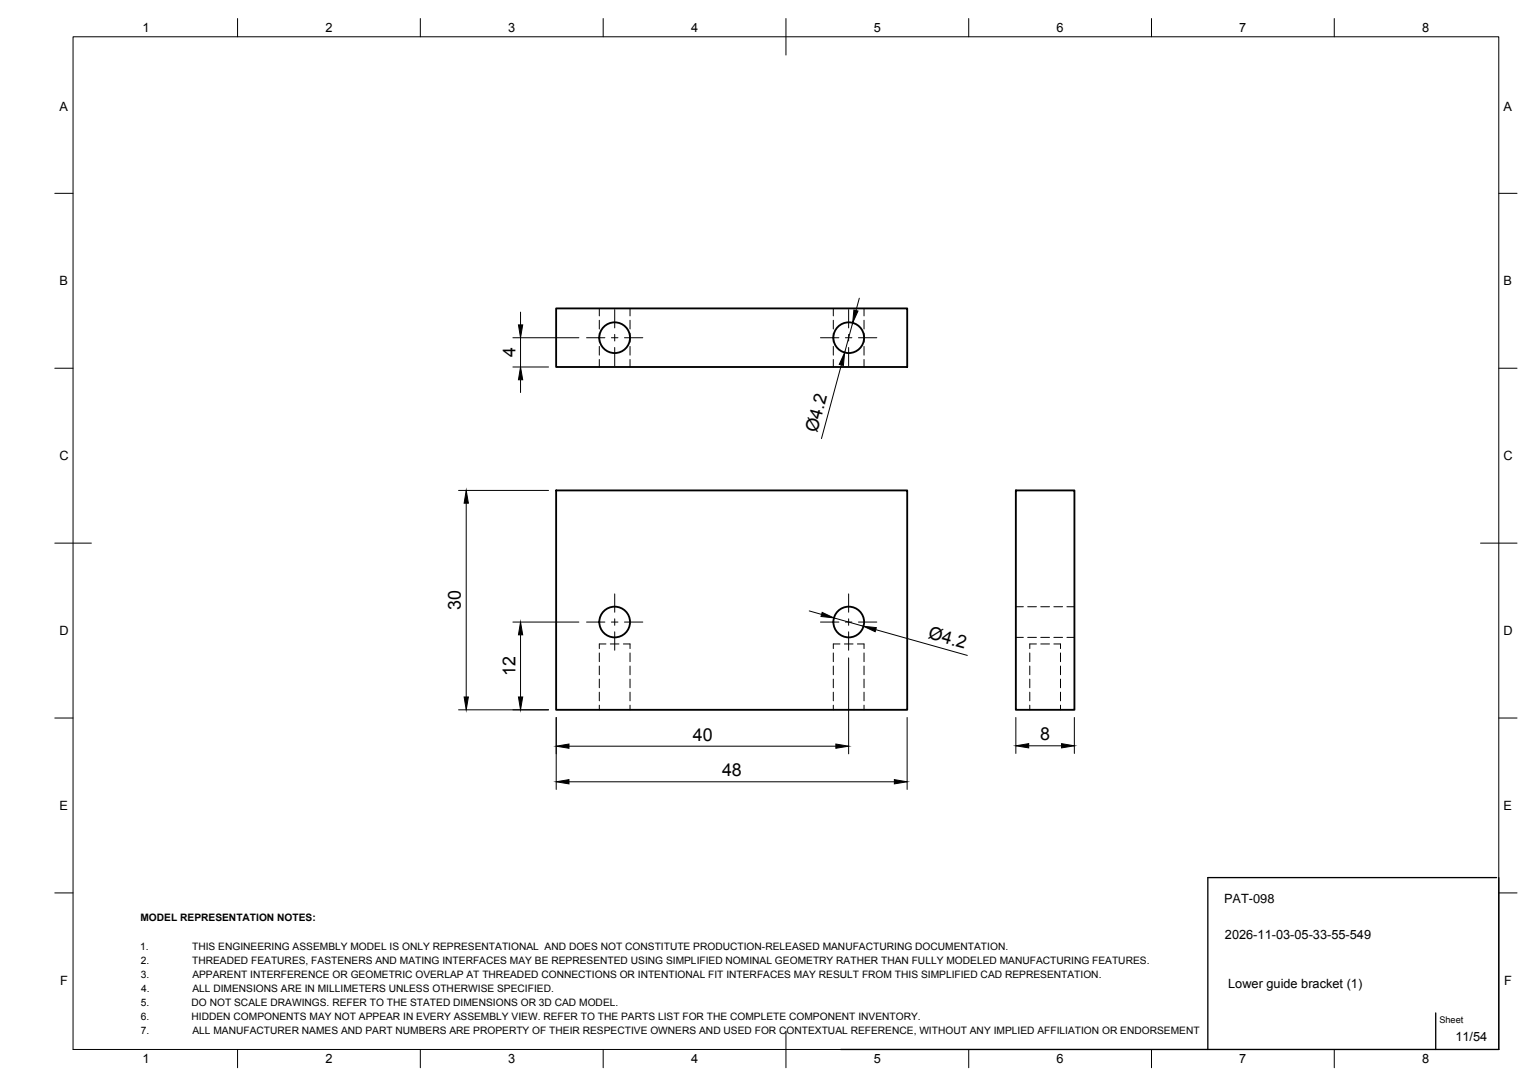
ISO-10303-21;
HEADER;
/* Generated by software containing ST-Developer
 * from STEP Tools, Inc. (www.steptools.com) 
 */

FILE_DESCRIPTION(
/* description */ ('Spring compression tester'),
/* implementation_level */ '2;1');

FILE_NAME(
/* name */ 'Lower guide bracket (1).step',
/* time_stamp */ '2026-10-28T03:24:11-07:00',
/* author */ (''),
/* organization */ (''),
/* preprocessor_version */ 'ST-DEVELOPER v20.2',
/* originating_system */ 'Autodesk Translation Framework v15.17.0.0',
/* authorisation */ '');

FILE_SCHEMA (('AUTOMOTIVE_DESIGN { 1 0 10303 214 3 1 1 }'));
ENDSEC;

DATA;
#10=MECHANICAL_DESIGN_GEOMETRIC_PRESENTATION_REPRESENTATION('',(#1112),#43521);
#992=SHAPE_REPRESENTATION_RELATIONSHIP('SRR','None',#43804,#1052);
#1052=ADVANCED_BREP_SHAPE_REPRESENTATION('',(#1187),#43464);
#1112=STYLED_ITEM('',(#44181),#1187);
#1187=MANIFOLD_SOLID_BREP('Body1',#18549);
#1333=FACE_BOUND('',#3434,.T.);
#1334=FACE_BOUND('',#3435,.T.);
#1335=FACE_BOUND('',#3438,.T.);
#1336=FACE_BOUND('',#3439,.T.);
#1337=FACE_BOUND('',#3443,.T.);
#1338=FACE_BOUND('',#3444,.T.);
#1663=PLANE('',#19526);
#1664=PLANE('',#19530);
#1665=PLANE('',#19537);
#1666=PLANE('',#19538);
#1667=PLANE('',#19539);
#1668=PLANE('',#19540);
#1669=PLANE('',#19541);
#1670=PLANE('',#19542);
#2294=FACE_OUTER_BOUND('',#3427,.T.);
#2295=FACE_OUTER_BOUND('',#3428,.T.);
#2296=FACE_OUTER_BOUND('',#3429,.T.);
#2297=FACE_OUTER_BOUND('',#3430,.T.);
#2298=FACE_OUTER_BOUND('',#3431,.T.);
#2299=FACE_OUTER_BOUND('',#3432,.T.);
#2300=FACE_OUTER_BOUND('',#3433,.T.);
#2301=FACE_OUTER_BOUND('',#3436,.T.);
#2302=FACE_OUTER_BOUND('',#3437,.T.);
#2303=FACE_OUTER_BOUND('',#3440,.T.);
#2304=FACE_OUTER_BOUND('',#3441,.T.);
#2305=FACE_OUTER_BOUND('',#3442,.T.);
#3427=EDGE_LOOP('',(#12793,#12794,#12795,#12796));
#3428=EDGE_LOOP('',(#12797));
#3429=EDGE_LOOP('',(#12798,#12799,#12800,#12801));
#3430=EDGE_LOOP('',(#12802));
#3431=EDGE_LOOP('',(#12803,#12804,#12805,#12806));
#3432=EDGE_LOOP('',(#12807,#12808,#12809,#12810));
#3433=EDGE_LOOP('',(#12811,#12812,#12813,#12814));
#3434=EDGE_LOOP('',(#12815));
#3435=EDGE_LOOP('',(#12816));
#3436=EDGE_LOOP('',(#12817,#12818,#12819,#12820));
#3437=EDGE_LOOP('',(#12821,#12822,#12823,#12824));
#3438=EDGE_LOOP('',(#12825));
#3439=EDGE_LOOP('',(#12826));
#3440=EDGE_LOOP('',(#12827,#12828,#12829,#12830));
#3441=EDGE_LOOP('',(#12831,#12832,#12833,#12834));
#3442=EDGE_LOOP('',(#12835,#12836,#12837,#12838));
#3443=EDGE_LOOP('',(#12839));
#3444=EDGE_LOOP('',(#12840));
#4790=LINE('',#27071,#6222);
#4791=LINE('',#27078,#6223);
#4792=LINE('',#27085,#6224);
#4793=LINE('',#27091,#6225);
#4794=LINE('',#27096,#6226);
#4795=LINE('',#27098,#6227);
#4796=LINE('',#27100,#6228);
#4797=LINE('',#27101,#6229);
#4798=LINE('',#27104,#6230);
#4799=LINE('',#27106,#6231);
#4800=LINE('',#27107,#6232);
#4801=LINE('',#27110,#6233);
#4802=LINE('',#27112,#6234);
#4803=LINE('',#27113,#6235);
#4804=LINE('',#27115,#6236);
#4805=LINE('',#27116,#6237);
#6222=VECTOR('',#21862,0.21);
#6223=VECTOR('',#21871,0.21);
#6224=VECTOR('',#21880,0.21);
#6225=VECTOR('',#21887,0.21);
#6226=VECTOR('',#21892,1.);
#6227=VECTOR('',#21893,1.);
#6228=VECTOR('',#21894,1.);
#6229=VECTOR('',#21895,1.);
#6230=VECTOR('',#21898,1.);
#6231=VECTOR('',#21899,1.);
#6232=VECTOR('',#21900,1.);
#6233=VECTOR('',#21903,1.);
#6234=VECTOR('',#21904,1.);
#6235=VECTOR('',#21905,1.);
#6236=VECTOR('',#21908,1.);
#6237=VECTOR('',#21909,1.);
#7574=CIRCLE('',#19524,0.21);
#7575=CIRCLE('',#19525,0.21);
#7576=CIRCLE('',#19528,0.21);
#7577=CIRCLE('',#19529,0.21);
#7578=CIRCLE('',#19532,0.21);
#7579=CIRCLE('',#19533,0.21);
#7580=CIRCLE('',#19535,0.21);
#7581=CIRCLE('',#19536,0.21);
#8328=VERTEX_POINT('',#27068);
#8329=VERTEX_POINT('',#27070);
#8330=VERTEX_POINT('',#27075);
#8331=VERTEX_POINT('',#27077);
#8332=VERTEX_POINT('',#27082);
#8333=VERTEX_POINT('',#27084);
#8334=VERTEX_POINT('',#27088);
#8335=VERTEX_POINT('',#27090);
#8336=VERTEX_POINT('',#27094);
#8337=VERTEX_POINT('',#27095);
#8338=VERTEX_POINT('',#27097);
#8339=VERTEX_POINT('',#27099);
#8340=VERTEX_POINT('',#27103);
#8341=VERTEX_POINT('',#27105);
#8342=VERTEX_POINT('',#27109);
#8343=VERTEX_POINT('',#27111);
#10061=EDGE_CURVE('',#8328,#8328,#7574,.T.);
#10062=EDGE_CURVE('',#8328,#8329,#4790,.T.);
#10063=EDGE_CURVE('',#8329,#8329,#7575,.T.);
#10064=EDGE_CURVE('',#8330,#8330,#7576,.T.);
#10065=EDGE_CURVE('',#8330,#8331,#4791,.T.);
#10066=EDGE_CURVE('',#8331,#8331,#7577,.T.);
#10067=EDGE_CURVE('',#8332,#8332,#7578,.T.);
#10068=EDGE_CURVE('',#8332,#8333,#4792,.T.);
#10069=EDGE_CURVE('',#8333,#8333,#7579,.T.);
#10070=EDGE_CURVE('',#8334,#8334,#7580,.T.);
#10071=EDGE_CURVE('',#8334,#8335,#4793,.T.);
#10072=EDGE_CURVE('',#8335,#8335,#7581,.T.);
#10073=EDGE_CURVE('',#8336,#8337,#4794,.T.);
#10074=EDGE_CURVE('',#8337,#8338,#4795,.T.);
#10075=EDGE_CURVE('',#8339,#8338,#4796,.T.);
#10076=EDGE_CURVE('',#8336,#8339,#4797,.T.);
#10077=EDGE_CURVE('',#8340,#8336,#4798,.T.);
#10078=EDGE_CURVE('',#8341,#8339,#4799,.T.);
#10079=EDGE_CURVE('',#8340,#8341,#4800,.T.);
#10080=EDGE_CURVE('',#8342,#8340,#4801,.T.);
#10081=EDGE_CURVE('',#8343,#8341,#4802,.T.);
#10082=EDGE_CURVE('',#8342,#8343,#4803,.T.);
#10083=EDGE_CURVE('',#8337,#8342,#4804,.T.);
#10084=EDGE_CURVE('',#8338,#8343,#4805,.T.);
#12793=ORIENTED_EDGE('',*,*,#10061,.F.);
#12794=ORIENTED_EDGE('',*,*,#10062,.T.);
#12795=ORIENTED_EDGE('',*,*,#10063,.T.);
#12796=ORIENTED_EDGE('',*,*,#10062,.F.);
#12797=ORIENTED_EDGE('',*,*,#10063,.F.);
#12798=ORIENTED_EDGE('',*,*,#10064,.F.);
#12799=ORIENTED_EDGE('',*,*,#10065,.T.);
#12800=ORIENTED_EDGE('',*,*,#10066,.T.);
#12801=ORIENTED_EDGE('',*,*,#10065,.F.);
#12802=ORIENTED_EDGE('',*,*,#10066,.F.);
#12803=ORIENTED_EDGE('',*,*,#10067,.F.);
#12804=ORIENTED_EDGE('',*,*,#10068,.T.);
#12805=ORIENTED_EDGE('',*,*,#10069,.F.);
#12806=ORIENTED_EDGE('',*,*,#10068,.F.);
#12807=ORIENTED_EDGE('',*,*,#10070,.F.);
#12808=ORIENTED_EDGE('',*,*,#10071,.T.);
#12809=ORIENTED_EDGE('',*,*,#10072,.F.);
#12810=ORIENTED_EDGE('',*,*,#10071,.F.);
#12811=ORIENTED_EDGE('',*,*,#10073,.T.);
#12812=ORIENTED_EDGE('',*,*,#10074,.T.);
#12813=ORIENTED_EDGE('',*,*,#10075,.F.);
#12814=ORIENTED_EDGE('',*,*,#10076,.F.);
#12815=ORIENTED_EDGE('',*,*,#10069,.T.);
#12816=ORIENTED_EDGE('',*,*,#10072,.T.);
#12817=ORIENTED_EDGE('',*,*,#10077,.T.);
#12818=ORIENTED_EDGE('',*,*,#10076,.T.);
#12819=ORIENTED_EDGE('',*,*,#10078,.F.);
#12820=ORIENTED_EDGE('',*,*,#10079,.F.);
#12821=ORIENTED_EDGE('',*,*,#10080,.T.);
#12822=ORIENTED_EDGE('',*,*,#10079,.T.);
#12823=ORIENTED_EDGE('',*,*,#10081,.F.);
#12824=ORIENTED_EDGE('',*,*,#10082,.F.);
#12825=ORIENTED_EDGE('',*,*,#10067,.T.);
#12826=ORIENTED_EDGE('',*,*,#10070,.T.);
#12827=ORIENTED_EDGE('',*,*,#10083,.T.);
#12828=ORIENTED_EDGE('',*,*,#10082,.T.);
#12829=ORIENTED_EDGE('',*,*,#10084,.F.);
#12830=ORIENTED_EDGE('',*,*,#10074,.F.);
#12831=ORIENTED_EDGE('',*,*,#10084,.T.);
#12832=ORIENTED_EDGE('',*,*,#10081,.T.);
#12833=ORIENTED_EDGE('',*,*,#10078,.T.);
#12834=ORIENTED_EDGE('',*,*,#10075,.T.);
#12835=ORIENTED_EDGE('',*,*,#10083,.F.);
#12836=ORIENTED_EDGE('',*,*,#10073,.F.);
#12837=ORIENTED_EDGE('',*,*,#10077,.F.);
#12838=ORIENTED_EDGE('',*,*,#10080,.F.);
#12839=ORIENTED_EDGE('',*,*,#10061,.T.);
#12840=ORIENTED_EDGE('',*,*,#10064,.T.);
#17155=CYLINDRICAL_SURFACE('',#19523,0.21);
#17156=CYLINDRICAL_SURFACE('',#19527,0.21);
#17157=CYLINDRICAL_SURFACE('',#19531,0.21);
#17158=CYLINDRICAL_SURFACE('',#19534,0.21);
#17618=ADVANCED_FACE('',(#2294),#17155,.F.);
#17619=ADVANCED_FACE('',(#2295),#1663,.F.);
#17620=ADVANCED_FACE('',(#2296),#17156,.F.);
#17621=ADVANCED_FACE('',(#2297),#1664,.F.);
#17622=ADVANCED_FACE('',(#2298),#17157,.F.);
#17623=ADVANCED_FACE('',(#2299),#17158,.F.);
#17624=ADVANCED_FACE('',(#2300,#1333,#1334),#1665,.T.);
#17625=ADVANCED_FACE('',(#2301),#1666,.T.);
#17626=ADVANCED_FACE('',(#2302,#1335,#1336),#1667,.T.);
#17627=ADVANCED_FACE('',(#2303),#1668,.T.);
#17628=ADVANCED_FACE('',(#2304),#1669,.T.);
#17629=ADVANCED_FACE('',(#2305,#1337,#1338),#1670,.F.);
#18549=CLOSED_SHELL('',(#17618,#17619,#17620,#17621,#17622,#17623,#17624,
#17625,#17626,#17627,#17628,#17629));
#19522=AXIS2_PLACEMENT_3D('',#27066,#21856,#21857);
#19523=AXIS2_PLACEMENT_3D('',#27067,#21858,#21859);
#19524=AXIS2_PLACEMENT_3D('',#27069,#21860,#21861);
#19525=AXIS2_PLACEMENT_3D('',#27072,#21863,#21864);
#19526=AXIS2_PLACEMENT_3D('',#27073,#21865,#21866);
#19527=AXIS2_PLACEMENT_3D('',#27074,#21867,#21868);
#19528=AXIS2_PLACEMENT_3D('',#27076,#21869,#21870);
#19529=AXIS2_PLACEMENT_3D('',#27079,#21872,#21873);
#19530=AXIS2_PLACEMENT_3D('',#27080,#21874,#21875);
#19531=AXIS2_PLACEMENT_3D('',#27081,#21876,#21877);
#19532=AXIS2_PLACEMENT_3D('',#27083,#21878,#21879);
#19533=AXIS2_PLACEMENT_3D('',#27086,#21881,#21882);
#19534=AXIS2_PLACEMENT_3D('',#27087,#21883,#21884);
#19535=AXIS2_PLACEMENT_3D('',#27089,#21885,#21886);
#19536=AXIS2_PLACEMENT_3D('',#27092,#21888,#21889);
#19537=AXIS2_PLACEMENT_3D('',#27093,#21890,#21891);
#19538=AXIS2_PLACEMENT_3D('',#27102,#21896,#21897);
#19539=AXIS2_PLACEMENT_3D('',#27108,#21901,#21902);
#19540=AXIS2_PLACEMENT_3D('',#27114,#21906,#21907);
#19541=AXIS2_PLACEMENT_3D('',#27117,#21910,#21911);
#19542=AXIS2_PLACEMENT_3D('',#27118,#21912,#21913);
#21856=DIRECTION('axis',(0.,0.,1.));
#21857=DIRECTION('refdir',(1.,0.,0.));
#21858=DIRECTION('center_axis',(0.,0.,1.));
#21859=DIRECTION('ref_axis',(1.,0.,0.));
#21860=DIRECTION('center_axis',(0.,0.,1.));
#21861=DIRECTION('ref_axis',(1.,0.,0.));
#21862=DIRECTION('',(0.,0.,1.));
#21863=DIRECTION('center_axis',(0.,0.,1.));
#21864=DIRECTION('ref_axis',(1.,0.,0.));
#21865=DIRECTION('center_axis',(0.,0.,1.));
#21866=DIRECTION('ref_axis',(1.,0.,0.));
#21867=DIRECTION('center_axis',(0.,0.,1.));
#21868=DIRECTION('ref_axis',(1.,0.,0.));
#21869=DIRECTION('center_axis',(0.,0.,1.));
#21870=DIRECTION('ref_axis',(1.,0.,0.));
#21871=DIRECTION('',(0.,0.,1.));
#21872=DIRECTION('center_axis',(0.,0.,1.));
#21873=DIRECTION('ref_axis',(1.,0.,0.));
#21874=DIRECTION('center_axis',(0.,0.,1.));
#21875=DIRECTION('ref_axis',(1.,0.,0.));
#21876=DIRECTION('center_axis',(0.,1.,0.));
#21877=DIRECTION('ref_axis',(1.,0.,0.));
#21878=DIRECTION('center_axis',(0.,1.,0.));
#21879=DIRECTION('ref_axis',(1.,0.,0.));
#21880=DIRECTION('',(0.,1.,0.));
#21881=DIRECTION('center_axis',(0.,-1.,0.));
#21882=DIRECTION('ref_axis',(1.,0.,0.));
#21883=DIRECTION('center_axis',(0.,1.,0.));
#21884=DIRECTION('ref_axis',(1.,0.,0.));
#21885=DIRECTION('center_axis',(0.,1.,0.));
#21886=DIRECTION('ref_axis',(1.,0.,0.));
#21887=DIRECTION('',(0.,1.,0.));
#21888=DIRECTION('center_axis',(0.,-1.,0.));
#21889=DIRECTION('ref_axis',(1.,0.,0.));
#21890=DIRECTION('center_axis',(0.,1.,0.));
#21891=DIRECTION('ref_axis',(-1.,0.,0.));
#21892=DIRECTION('',(-1.,0.,0.));
#21893=DIRECTION('',(0.,0.,1.));
#21894=DIRECTION('',(-1.,0.,0.));
#21895=DIRECTION('',(0.,0.,1.));
#21896=DIRECTION('center_axis',(1.,0.,0.));
#21897=DIRECTION('ref_axis',(0.,1.,0.));
#21898=DIRECTION('',(0.,1.,0.));
#21899=DIRECTION('',(0.,1.,0.));
#21900=DIRECTION('',(0.,0.,1.));
#21901=DIRECTION('center_axis',(0.,-1.,0.));
#21902=DIRECTION('ref_axis',(1.,0.,0.));
#21903=DIRECTION('',(1.,0.,0.));
#21904=DIRECTION('',(1.,0.,0.));
#21905=DIRECTION('',(0.,0.,1.));
#21906=DIRECTION('center_axis',(-1.,0.,0.));
#21907=DIRECTION('ref_axis',(0.,-1.,0.));
#21908=DIRECTION('',(0.,-1.,0.));
#21909=DIRECTION('',(0.,-1.,0.));
#21910=DIRECTION('center_axis',(0.,0.,1.));
#21911=DIRECTION('ref_axis',(1.,0.,0.));
#21912=DIRECTION('center_axis',(0.,0.,1.));
#21913=DIRECTION('ref_axis',(1.,0.,0.));
#27066=CARTESIAN_POINT('',(0.,0.,0.));
#27067=CARTESIAN_POINT('Origin',(4.4,2.7,-0.1));
#27068=CARTESIAN_POINT('',(4.19,2.7,0.));
#27069=CARTESIAN_POINT('Origin',(4.4,2.7,0.));
#27070=CARTESIAN_POINT('',(4.19,2.7,0.9));
#27071=CARTESIAN_POINT('',(4.19,2.7,-0.1));
#27072=CARTESIAN_POINT('Origin',(4.4,2.7,0.9));
#27073=CARTESIAN_POINT('Origin',(4.4,2.7,0.9));
#27074=CARTESIAN_POINT('Origin',(7.6,2.7,-0.1));
#27075=CARTESIAN_POINT('',(7.39,2.7,0.));
#27076=CARTESIAN_POINT('Origin',(7.6,2.7,0.));
#27077=CARTESIAN_POINT('',(7.39,2.7,0.9));
#27078=CARTESIAN_POINT('',(7.39,2.7,-0.1));
#27079=CARTESIAN_POINT('Origin',(7.6,2.7,0.9));
#27080=CARTESIAN_POINT('Origin',(7.6,2.7,0.9));
#27081=CARTESIAN_POINT('Origin',(4.4,2.2,1.2));
#27082=CARTESIAN_POINT('',(4.19,2.3,1.2));
#27083=CARTESIAN_POINT('Origin',(4.4,2.3,1.2));
#27084=CARTESIAN_POINT('',(4.19,3.1,1.2));
#27085=CARTESIAN_POINT('',(4.19,2.2,1.2));
#27086=CARTESIAN_POINT('Origin',(4.4,3.1,1.2));
#27087=CARTESIAN_POINT('Origin',(7.6,2.2,1.2));
#27088=CARTESIAN_POINT('',(7.39,2.3,1.2));
#27089=CARTESIAN_POINT('Origin',(7.6,2.3,1.2));
#27090=CARTESIAN_POINT('',(7.39,3.1,1.2));
#27091=CARTESIAN_POINT('',(7.39,2.2,1.2));
#27092=CARTESIAN_POINT('Origin',(7.6,3.1,1.2));
#27093=CARTESIAN_POINT('Origin',(8.4,3.1,0.));
#27094=CARTESIAN_POINT('',(8.4,3.1,0.));
#27095=CARTESIAN_POINT('',(3.6,3.1,0.));
#27096=CARTESIAN_POINT('',(8.4,3.1,0.));
#27097=CARTESIAN_POINT('',(3.6,3.1,3.));
#27098=CARTESIAN_POINT('',(3.6,3.1,0.));
#27099=CARTESIAN_POINT('',(8.4,3.1,3.));
#27100=CARTESIAN_POINT('',(8.4,3.1,3.));
#27101=CARTESIAN_POINT('',(8.4,3.1,0.));
#27102=CARTESIAN_POINT('Origin',(8.4,2.3,0.));
#27103=CARTESIAN_POINT('',(8.4,2.3,0.));
#27104=CARTESIAN_POINT('',(8.4,2.3,0.));
#27105=CARTESIAN_POINT('',(8.4,2.3,3.));
#27106=CARTESIAN_POINT('',(8.4,2.3,3.));
#27107=CARTESIAN_POINT('',(8.4,2.3,0.));
#27108=CARTESIAN_POINT('Origin',(3.6,2.3,0.));
#27109=CARTESIAN_POINT('',(3.6,2.3,0.));
#27110=CARTESIAN_POINT('',(3.6,2.3,0.));
#27111=CARTESIAN_POINT('',(3.6,2.3,3.));
#27112=CARTESIAN_POINT('',(3.6,2.3,3.));
#27113=CARTESIAN_POINT('',(3.6,2.3,0.));
#27114=CARTESIAN_POINT('Origin',(3.6,3.1,0.));
#27115=CARTESIAN_POINT('',(3.6,3.1,0.));
#27116=CARTESIAN_POINT('',(3.6,3.1,3.));
#27117=CARTESIAN_POINT('Origin',(6.,2.7,3.));
#27118=CARTESIAN_POINT('Origin',(6.,2.7,0.));
#43396=UNCERTAINTY_MEASURE_WITH_UNIT(LENGTH_MEASURE(0.001),#43522,
'DISTANCE_ACCURACY_VALUE',
'Maximum model space distance between geometric entities at asserted c
onnectivities');
#43453=UNCERTAINTY_MEASURE_WITH_UNIT(LENGTH_MEASURE(0.001),#43522,
'DISTANCE_ACCURACY_VALUE',
'Maximum model space distance between geometric entities at asserted c
onnectivities');
#43464=(
GEOMETRIC_REPRESENTATION_CONTEXT(3)
GLOBAL_UNCERTAINTY_ASSIGNED_CONTEXT((#43396))
GLOBAL_UNIT_ASSIGNED_CONTEXT((#43522,#43524,#43525))
REPRESENTATION_CONTEXT('','3D')
);
#43521=(
GEOMETRIC_REPRESENTATION_CONTEXT(3)
GLOBAL_UNCERTAINTY_ASSIGNED_CONTEXT((#43453))
GLOBAL_UNIT_ASSIGNED_CONTEXT((#43522,#43524,#43525))
REPRESENTATION_CONTEXT('','3D')
);
#43522=(
LENGTH_UNIT()
NAMED_UNIT(*)
SI_UNIT(.CENTI.,.METRE.)
);
#43524=(
NAMED_UNIT(*)
PLANE_ANGLE_UNIT()
SI_UNIT($,.RADIAN.)
);
#43525=(
NAMED_UNIT(*)
SI_UNIT($,.STERADIAN.)
SOLID_ANGLE_UNIT()
);
#43536=SHAPE_DEFINITION_REPRESENTATION(#43603,#43804);
#43603=PRODUCT_DEFINITION_SHAPE('',$,#43872);
#43804=SHAPE_REPRESENTATION('',(#19522),#43464);
#43861=PRODUCT_DEFINITION_CONTEXT('part definition',#44064,'design');
#43872=PRODUCT_DEFINITION('Lower guide bracket (1)',
'Lower guide bracket (1)',#43939,#43861);
#43939=PRODUCT_DEFINITION_FORMATION('',$,#44076);
#44064=APPLICATION_CONTEXT(
'Core Data for Automotive Mechanical Design Process');
#44065=PRODUCT_CONTEXT('part definition',#44064,'mechanical');
#44076=PRODUCT('Lower guide bracket (1)','Lower guide bracket (1)',
'Lower guide bracket (1)',(#44065));
#44175=COLOUR_RGB('Dark Blue',0.08,0.2,0.34);
#44176=FILL_AREA_STYLE_COLOUR('',#44175);
#44177=FILL_AREA_STYLE('',(#44176));
#44178=SURFACE_STYLE_FILL_AREA(#44177);
#44179=SURFACE_SIDE_STYLE('',(#44178));
#44180=SURFACE_STYLE_USAGE(.BOTH.,#44179);
#44181=PRESENTATION_STYLE_ASSIGNMENT((#44180));
ENDSEC;
END-ISO-10303-21;
